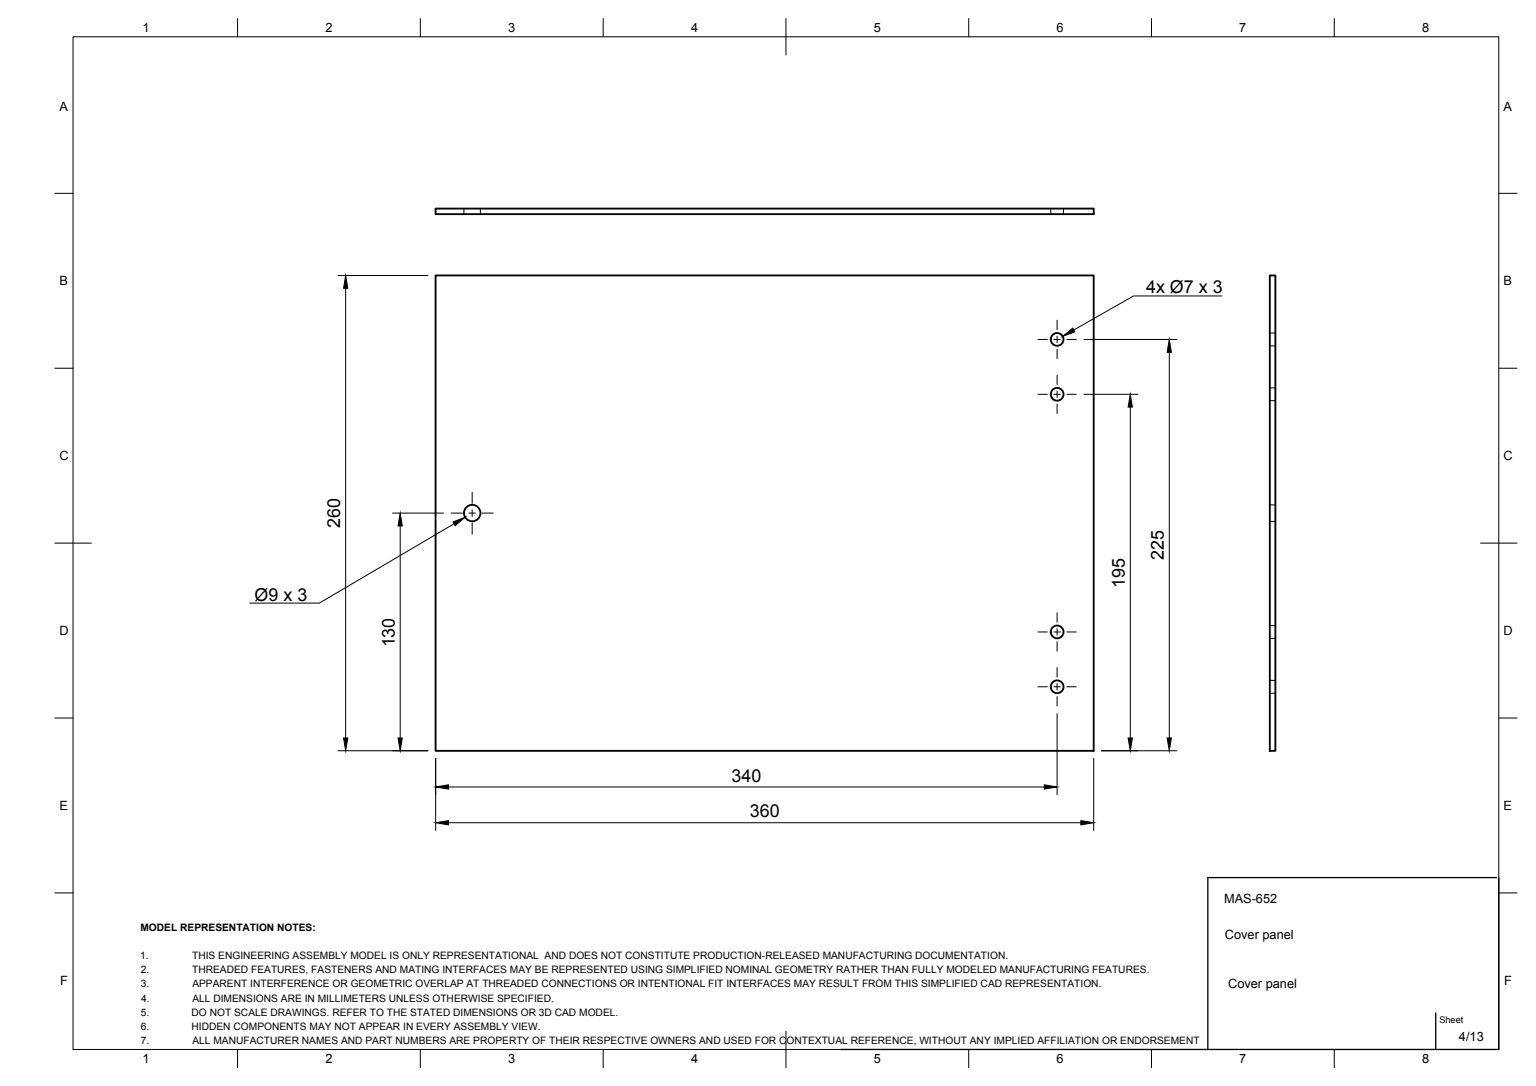
ISO-10303-21;
HEADER;
/* Generated by software containing ST-Developer
 * from STEP Tools, Inc. (www.steptools.com) 
 */

FILE_DESCRIPTION(
/* description */ ('Independent hinged machine back cover with retained hinge pins, perim
eter gasket and quarter-turn cam latch. Nominal cover 360 x 260 x 3 mm
, frame 430 x 300 x 20 mm. No guarding, structural or ingress rating a
ssigned.'),
/* implementation_level */ '2;1');

FILE_NAME(
/* name */ 'Cover panel.step',
/* time_stamp */ '2026-11-09T19:36:59-08:00',
/* author */ (''),
/* organization */ (''),
/* preprocessor_version */ 'ST-DEVELOPER v20.2',
/* originating_system */ 'Autodesk Translation Framework v15.17.0.0',
/* authorisation */ '');

FILE_SCHEMA (('AUTOMOTIVE_DESIGN { 1 0 10303 214 3 1 1 }'));
ENDSEC;

DATA;
#10=MECHANICAL_DESIGN_GEOMETRIC_PRESENTATION_REPRESENTATION('',(#199),#32627);
#163=SHAPE_REPRESENTATION_RELATIONSHIP('SRR','None',#32709,#181);
#181=ADVANCED_BREP_SHAPE_REPRESENTATION('',(#217),#32610);
#199=STYLED_ITEM('',(#32808),#217);
#217=MANIFOLD_SOLID_BREP('Body1',#8676);
#240=FACE_BOUND('',#1113,.T.);
#241=FACE_BOUND('',#1114,.T.);
#242=FACE_BOUND('',#1115,.T.);
#243=FACE_BOUND('',#1116,.T.);
#244=FACE_BOUND('',#1117,.T.);
#245=FACE_BOUND('',#1119,.T.);
#246=FACE_BOUND('',#1120,.T.);
#247=FACE_BOUND('',#1121,.T.);
#248=FACE_BOUND('',#1122,.T.);
#249=FACE_BOUND('',#1123,.T.);
#329=PLANE('',#9096);
#330=PLANE('',#9097);
#331=PLANE('',#9098);
#332=PLANE('',#9099);
#333=PLANE('',#9100);
#334=PLANE('',#9101);
#622=FACE_OUTER_BOUND('',#1103,.T.);
#623=FACE_OUTER_BOUND('',#1104,.T.);
#624=FACE_OUTER_BOUND('',#1105,.T.);
#625=FACE_OUTER_BOUND('',#1106,.T.);
#626=FACE_OUTER_BOUND('',#1107,.T.);
#627=FACE_OUTER_BOUND('',#1108,.T.);
#628=FACE_OUTER_BOUND('',#1109,.T.);
#629=FACE_OUTER_BOUND('',#1110,.T.);
#630=FACE_OUTER_BOUND('',#1111,.T.);
#631=FACE_OUTER_BOUND('',#1112,.T.);
#632=FACE_OUTER_BOUND('',#1118,.T.);
#1103=EDGE_LOOP('',(#6351,#6352,#6353,#6354));
#1104=EDGE_LOOP('',(#6355,#6356,#6357,#6358));
#1105=EDGE_LOOP('',(#6359,#6360,#6361,#6362));
#1106=EDGE_LOOP('',(#6363,#6364,#6365,#6366));
#1107=EDGE_LOOP('',(#6367,#6368,#6369,#6370));
#1108=EDGE_LOOP('',(#6371,#6372,#6373,#6374));
#1109=EDGE_LOOP('',(#6375,#6376,#6377,#6378));
#1110=EDGE_LOOP('',(#6379,#6380,#6381,#6382));
#1111=EDGE_LOOP('',(#6383,#6384,#6385,#6386));
#1112=EDGE_LOOP('',(#6387,#6388,#6389,#6390));
#1113=EDGE_LOOP('',(#6391));
#1114=EDGE_LOOP('',(#6392));
#1115=EDGE_LOOP('',(#6393));
#1116=EDGE_LOOP('',(#6394));
#1117=EDGE_LOOP('',(#6395));
#1118=EDGE_LOOP('',(#6396,#6397,#6398,#6399));
#1119=EDGE_LOOP('',(#6400));
#1120=EDGE_LOOP('',(#6401));
#1121=EDGE_LOOP('',(#6402));
#1122=EDGE_LOOP('',(#6403));
#1123=EDGE_LOOP('',(#6404));
#1485=CIRCLE('',#9082,4.5);
#1486=CIRCLE('',#9083,4.5);
#1487=CIRCLE('',#9085,3.5);
#1488=CIRCLE('',#9086,3.5);
#1489=CIRCLE('',#9088,3.5);
#1490=CIRCLE('',#9089,3.5);
#1491=CIRCLE('',#9091,3.5);
#1492=CIRCLE('',#9092,3.5);
#1493=CIRCLE('',#9094,3.5);
#1494=CIRCLE('',#9095,3.5);
#2339=LINE('',#21642,#2885);
#2340=LINE('',#21648,#2886);
#2341=LINE('',#21654,#2887);
#2342=LINE('',#21660,#2888);
#2343=LINE('',#21666,#2889);
#2344=LINE('',#21671,#2890);
#2345=LINE('',#21673,#2891);
#2346=LINE('',#21675,#2892);
#2347=LINE('',#21676,#2893);
#2348=LINE('',#21679,#2894);
#2349=LINE('',#21681,#2895);
#2350=LINE('',#21682,#2896);
#2351=LINE('',#21685,#2897);
#2352=LINE('',#21687,#2898);
#2353=LINE('',#21688,#2899);
#2354=LINE('',#21690,#2900);
#2355=LINE('',#21691,#2901);
#2885=VECTOR('',#10075,4.5);
#2886=VECTOR('',#10082,3.5);
#2887=VECTOR('',#10089,3.5);
#2888=VECTOR('',#10096,3.5);
#2889=VECTOR('',#10103,3.5);
#2890=VECTOR('',#10108,10.);
#2891=VECTOR('',#10109,10.);
#2892=VECTOR('',#10110,10.);
#2893=VECTOR('',#10111,10.);
#2894=VECTOR('',#10114,10.);
#2895=VECTOR('',#10115,10.);
#2896=VECTOR('',#10116,10.);
#2897=VECTOR('',#10119,10.);
#2898=VECTOR('',#10120,10.);
#2899=VECTOR('',#10121,10.);
#2900=VECTOR('',#10124,10.);
#2901=VECTOR('',#10125,10.);
#3595=VERTEX_POINT('',#21639);
#3596=VERTEX_POINT('',#21641);
#3597=VERTEX_POINT('',#21645);
#3598=VERTEX_POINT('',#21647);
#3599=VERTEX_POINT('',#21651);
#3600=VERTEX_POINT('',#21653);
#3601=VERTEX_POINT('',#21657);
#3602=VERTEX_POINT('',#21659);
#3603=VERTEX_POINT('',#21663);
#3604=VERTEX_POINT('',#21665);
#3605=VERTEX_POINT('',#21669);
#3606=VERTEX_POINT('',#21670);
#3607=VERTEX_POINT('',#21672);
#3608=VERTEX_POINT('',#21674);
#3609=VERTEX_POINT('',#21678);
#3610=VERTEX_POINT('',#21680);
#3611=VERTEX_POINT('',#21684);
#3612=VERTEX_POINT('',#21686);
#4599=EDGE_CURVE('',#3595,#3595,#1485,.T.);
#4600=EDGE_CURVE('',#3595,#3596,#2339,.T.);
#4601=EDGE_CURVE('',#3596,#3596,#1486,.T.);
#4602=EDGE_CURVE('',#3597,#3597,#1487,.T.);
#4603=EDGE_CURVE('',#3597,#3598,#2340,.T.);
#4604=EDGE_CURVE('',#3598,#3598,#1488,.T.);
#4605=EDGE_CURVE('',#3599,#3599,#1489,.T.);
#4606=EDGE_CURVE('',#3599,#3600,#2341,.T.);
#4607=EDGE_CURVE('',#3600,#3600,#1490,.T.);
#4608=EDGE_CURVE('',#3601,#3601,#1491,.T.);
#4609=EDGE_CURVE('',#3601,#3602,#2342,.T.);
#4610=EDGE_CURVE('',#3602,#3602,#1492,.T.);
#4611=EDGE_CURVE('',#3603,#3603,#1493,.T.);
#4612=EDGE_CURVE('',#3603,#3604,#2343,.T.);
#4613=EDGE_CURVE('',#3604,#3604,#1494,.T.);
#4614=EDGE_CURVE('',#3605,#3606,#2344,.T.);
#4615=EDGE_CURVE('',#3606,#3607,#2345,.T.);
#4616=EDGE_CURVE('',#3608,#3607,#2346,.T.);
#4617=EDGE_CURVE('',#3605,#3608,#2347,.T.);
#4618=EDGE_CURVE('',#3609,#3605,#2348,.T.);
#4619=EDGE_CURVE('',#3610,#3608,#2349,.T.);
#4620=EDGE_CURVE('',#3609,#3610,#2350,.T.);
#4621=EDGE_CURVE('',#3611,#3609,#2351,.T.);
#4622=EDGE_CURVE('',#3612,#3610,#2352,.T.);
#4623=EDGE_CURVE('',#3611,#3612,#2353,.T.);
#4624=EDGE_CURVE('',#3606,#3611,#2354,.T.);
#4625=EDGE_CURVE('',#3607,#3612,#2355,.T.);
#6351=ORIENTED_EDGE('',*,*,#4599,.F.);
#6352=ORIENTED_EDGE('',*,*,#4600,.T.);
#6353=ORIENTED_EDGE('',*,*,#4601,.F.);
#6354=ORIENTED_EDGE('',*,*,#4600,.F.);
#6355=ORIENTED_EDGE('',*,*,#4602,.F.);
#6356=ORIENTED_EDGE('',*,*,#4603,.T.);
#6357=ORIENTED_EDGE('',*,*,#4604,.F.);
#6358=ORIENTED_EDGE('',*,*,#4603,.F.);
#6359=ORIENTED_EDGE('',*,*,#4605,.F.);
#6360=ORIENTED_EDGE('',*,*,#4606,.T.);
#6361=ORIENTED_EDGE('',*,*,#4607,.F.);
#6362=ORIENTED_EDGE('',*,*,#4606,.F.);
#6363=ORIENTED_EDGE('',*,*,#4608,.F.);
#6364=ORIENTED_EDGE('',*,*,#4609,.T.);
#6365=ORIENTED_EDGE('',*,*,#4610,.F.);
#6366=ORIENTED_EDGE('',*,*,#4609,.F.);
#6367=ORIENTED_EDGE('',*,*,#4611,.F.);
#6368=ORIENTED_EDGE('',*,*,#4612,.T.);
#6369=ORIENTED_EDGE('',*,*,#4613,.F.);
#6370=ORIENTED_EDGE('',*,*,#4612,.F.);
#6371=ORIENTED_EDGE('',*,*,#4614,.T.);
#6372=ORIENTED_EDGE('',*,*,#4615,.T.);
#6373=ORIENTED_EDGE('',*,*,#4616,.F.);
#6374=ORIENTED_EDGE('',*,*,#4617,.F.);
#6375=ORIENTED_EDGE('',*,*,#4618,.T.);
#6376=ORIENTED_EDGE('',*,*,#4617,.T.);
#6377=ORIENTED_EDGE('',*,*,#4619,.F.);
#6378=ORIENTED_EDGE('',*,*,#4620,.F.);
#6379=ORIENTED_EDGE('',*,*,#4621,.T.);
#6380=ORIENTED_EDGE('',*,*,#4620,.T.);
#6381=ORIENTED_EDGE('',*,*,#4622,.F.);
#6382=ORIENTED_EDGE('',*,*,#4623,.F.);
#6383=ORIENTED_EDGE('',*,*,#4624,.T.);
#6384=ORIENTED_EDGE('',*,*,#4623,.T.);
#6385=ORIENTED_EDGE('',*,*,#4625,.F.);
#6386=ORIENTED_EDGE('',*,*,#4615,.F.);
#6387=ORIENTED_EDGE('',*,*,#4625,.T.);
#6388=ORIENTED_EDGE('',*,*,#4622,.T.);
#6389=ORIENTED_EDGE('',*,*,#4619,.T.);
#6390=ORIENTED_EDGE('',*,*,#4616,.T.);
#6391=ORIENTED_EDGE('',*,*,#4599,.T.);
#6392=ORIENTED_EDGE('',*,*,#4602,.T.);
#6393=ORIENTED_EDGE('',*,*,#4605,.T.);
#6394=ORIENTED_EDGE('',*,*,#4608,.T.);
#6395=ORIENTED_EDGE('',*,*,#4611,.T.);
#6396=ORIENTED_EDGE('',*,*,#4624,.F.);
#6397=ORIENTED_EDGE('',*,*,#4614,.F.);
#6398=ORIENTED_EDGE('',*,*,#4618,.F.);
#6399=ORIENTED_EDGE('',*,*,#4621,.F.);
#6400=ORIENTED_EDGE('',*,*,#4601,.T.);
#6401=ORIENTED_EDGE('',*,*,#4604,.T.);
#6402=ORIENTED_EDGE('',*,*,#4607,.T.);
#6403=ORIENTED_EDGE('',*,*,#4610,.T.);
#6404=ORIENTED_EDGE('',*,*,#4613,.T.);
#8031=CYLINDRICAL_SURFACE('',#9081,4.5);
#8032=CYLINDRICAL_SURFACE('',#9084,3.5);
#8033=CYLINDRICAL_SURFACE('',#9087,3.5);
#8034=CYLINDRICAL_SURFACE('',#9090,3.5);
#8035=CYLINDRICAL_SURFACE('',#9093,3.5);
#8370=ADVANCED_FACE('',(#622),#8031,.F.);
#8371=ADVANCED_FACE('',(#623),#8032,.F.);
#8372=ADVANCED_FACE('',(#624),#8033,.F.);
#8373=ADVANCED_FACE('',(#625),#8034,.F.);
#8374=ADVANCED_FACE('',(#626),#8035,.F.);
#8375=ADVANCED_FACE('',(#627),#329,.T.);
#8376=ADVANCED_FACE('',(#628),#330,.T.);
#8377=ADVANCED_FACE('',(#629),#331,.T.);
#8378=ADVANCED_FACE('',(#630),#332,.T.);
#8379=ADVANCED_FACE('',(#631,#240,#241,#242,#243,#244),#333,.T.);
#8380=ADVANCED_FACE('',(#632,#245,#246,#247,#248,#249),#334,.F.);
#8676=CLOSED_SHELL('',(#8370,#8371,#8372,#8373,#8374,#8375,#8376,#8377,
#8378,#8379,#8380));
#9080=AXIS2_PLACEMENT_3D('',#21637,#10069,#10070);
#9081=AXIS2_PLACEMENT_3D('',#21638,#10071,#10072);
#9082=AXIS2_PLACEMENT_3D('',#21640,#10073,#10074);
#9083=AXIS2_PLACEMENT_3D('',#21643,#10076,#10077);
#9084=AXIS2_PLACEMENT_3D('',#21644,#10078,#10079);
#9085=AXIS2_PLACEMENT_3D('',#21646,#10080,#10081);
#9086=AXIS2_PLACEMENT_3D('',#21649,#10083,#10084);
#9087=AXIS2_PLACEMENT_3D('',#21650,#10085,#10086);
#9088=AXIS2_PLACEMENT_3D('',#21652,#10087,#10088);
#9089=AXIS2_PLACEMENT_3D('',#21655,#10090,#10091);
#9090=AXIS2_PLACEMENT_3D('',#21656,#10092,#10093);
#9091=AXIS2_PLACEMENT_3D('',#21658,#10094,#10095);
#9092=AXIS2_PLACEMENT_3D('',#21661,#10097,#10098);
#9093=AXIS2_PLACEMENT_3D('',#21662,#10099,#10100);
#9094=AXIS2_PLACEMENT_3D('',#21664,#10101,#10102);
#9095=AXIS2_PLACEMENT_3D('',#21667,#10104,#10105);
#9096=AXIS2_PLACEMENT_3D('',#21668,#10106,#10107);
#9097=AXIS2_PLACEMENT_3D('',#21677,#10112,#10113);
#9098=AXIS2_PLACEMENT_3D('',#21683,#10117,#10118);
#9099=AXIS2_PLACEMENT_3D('',#21689,#10122,#10123);
#9100=AXIS2_PLACEMENT_3D('',#21692,#10126,#10127);
#9101=AXIS2_PLACEMENT_3D('',#21693,#10128,#10129);
#10069=DIRECTION('axis',(0.,0.,1.));
#10070=DIRECTION('refdir',(1.,0.,0.));
#10071=DIRECTION('center_axis',(0.,0.,-1.));
#10072=DIRECTION('ref_axis',(1.,0.,0.));
#10073=DIRECTION('center_axis',(0.,0.,-1.));
#10074=DIRECTION('ref_axis',(1.,0.,0.));
#10075=DIRECTION('',(0.,0.,-1.));
#10076=DIRECTION('center_axis',(0.,0.,1.));
#10077=DIRECTION('ref_axis',(1.,0.,0.));
#10078=DIRECTION('center_axis',(0.,0.,-1.));
#10079=DIRECTION('ref_axis',(1.,0.,0.));
#10080=DIRECTION('center_axis',(0.,0.,-1.));
#10081=DIRECTION('ref_axis',(1.,0.,0.));
#10082=DIRECTION('',(0.,0.,-1.));
#10083=DIRECTION('center_axis',(0.,0.,1.));
#10084=DIRECTION('ref_axis',(1.,0.,0.));
#10085=DIRECTION('center_axis',(0.,0.,-1.));
#10086=DIRECTION('ref_axis',(1.,0.,0.));
#10087=DIRECTION('center_axis',(0.,0.,-1.));
#10088=DIRECTION('ref_axis',(1.,0.,0.));
#10089=DIRECTION('',(0.,0.,-1.));
#10090=DIRECTION('center_axis',(0.,0.,1.));
#10091=DIRECTION('ref_axis',(1.,0.,0.));
#10092=DIRECTION('center_axis',(0.,0.,-1.));
#10093=DIRECTION('ref_axis',(1.,0.,0.));
#10094=DIRECTION('center_axis',(0.,0.,-1.));
#10095=DIRECTION('ref_axis',(1.,0.,0.));
#10096=DIRECTION('',(0.,0.,-1.));
#10097=DIRECTION('center_axis',(0.,0.,1.));
#10098=DIRECTION('ref_axis',(1.,0.,0.));
#10099=DIRECTION('center_axis',(0.,0.,-1.));
#10100=DIRECTION('ref_axis',(1.,0.,0.));
#10101=DIRECTION('center_axis',(0.,0.,-1.));
#10102=DIRECTION('ref_axis',(1.,0.,0.));
#10103=DIRECTION('',(0.,0.,-1.));
#10104=DIRECTION('center_axis',(0.,0.,1.));
#10105=DIRECTION('ref_axis',(1.,0.,0.));
#10106=DIRECTION('center_axis',(0.,1.,0.));
#10107=DIRECTION('ref_axis',(-1.,0.,0.));
#10108=DIRECTION('',(-1.,0.,0.));
#10109=DIRECTION('',(0.,0.,1.));
#10110=DIRECTION('',(-1.,0.,0.));
#10111=DIRECTION('',(0.,0.,1.));
#10112=DIRECTION('center_axis',(1.,0.,0.));
#10113=DIRECTION('ref_axis',(0.,1.,0.));
#10114=DIRECTION('',(0.,1.,0.));
#10115=DIRECTION('',(0.,1.,0.));
#10116=DIRECTION('',(0.,0.,1.));
#10117=DIRECTION('center_axis',(0.,-1.,0.));
#10118=DIRECTION('ref_axis',(1.,0.,0.));
#10119=DIRECTION('',(1.,0.,0.));
#10120=DIRECTION('',(1.,0.,0.));
#10121=DIRECTION('',(0.,0.,1.));
#10122=DIRECTION('center_axis',(-1.,0.,0.));
#10123=DIRECTION('ref_axis',(0.,-1.,0.));
#10124=DIRECTION('',(0.,-1.,0.));
#10125=DIRECTION('',(0.,-1.,0.));
#10126=DIRECTION('center_axis',(0.,0.,1.));
#10127=DIRECTION('ref_axis',(1.,0.,0.));
#10128=DIRECTION('center_axis',(0.,0.,1.));
#10129=DIRECTION('ref_axis',(1.,0.,0.));
#21637=CARTESIAN_POINT('',(0.,0.,0.));
#21638=CARTESIAN_POINT('Origin',(160.,0.,1.5));
#21639=CARTESIAN_POINT('',(155.5,5.51091059616309E-16,3.));
#21640=CARTESIAN_POINT('Origin',(160.,0.,3.));
#21641=CARTESIAN_POINT('',(155.5,5.51091059616309E-16,0.));
#21642=CARTESIAN_POINT('',(155.5,5.51091059616309E-16,1.5));
#21643=CARTESIAN_POINT('Origin',(160.,0.,0.));
#21644=CARTESIAN_POINT('Origin',(-160.,65.,1.5));
#21645=CARTESIAN_POINT('',(-163.5,65.,3.));
#21646=CARTESIAN_POINT('Origin',(-160.,65.,3.));
#21647=CARTESIAN_POINT('',(-163.5,65.,0.));
#21648=CARTESIAN_POINT('',(-163.5,65.,1.5));
#21649=CARTESIAN_POINT('Origin',(-160.,65.,0.));
#21650=CARTESIAN_POINT('Origin',(-160.,-95.,1.5));
#21651=CARTESIAN_POINT('',(-163.5,-95.,3.));
#21652=CARTESIAN_POINT('Origin',(-160.,-95.,3.));
#21653=CARTESIAN_POINT('',(-163.5,-95.,0.));
#21654=CARTESIAN_POINT('',(-163.5,-95.,1.5));
#21655=CARTESIAN_POINT('Origin',(-160.,-95.,0.));
#21656=CARTESIAN_POINT('Origin',(-160.,-65.,1.5));
#21657=CARTESIAN_POINT('',(-163.5,-65.,3.));
#21658=CARTESIAN_POINT('Origin',(-160.,-65.,3.));
#21659=CARTESIAN_POINT('',(-163.5,-65.,0.));
#21660=CARTESIAN_POINT('',(-163.5,-65.,1.5));
#21661=CARTESIAN_POINT('Origin',(-160.,-65.,0.));
#21662=CARTESIAN_POINT('Origin',(-160.,95.,1.5));
#21663=CARTESIAN_POINT('',(-163.5,95.,3.));
#21664=CARTESIAN_POINT('Origin',(-160.,95.,3.));
#21665=CARTESIAN_POINT('',(-163.5,95.,0.));
#21666=CARTESIAN_POINT('',(-163.5,95.,1.5));
#21667=CARTESIAN_POINT('Origin',(-160.,95.,0.));
#21668=CARTESIAN_POINT('Origin',(180.,130.,0.));
#21669=CARTESIAN_POINT('',(180.,130.,0.));
#21670=CARTESIAN_POINT('',(-180.,130.,0.));
#21671=CARTESIAN_POINT('',(180.,130.,0.));
#21672=CARTESIAN_POINT('',(-180.,130.,3.));
#21673=CARTESIAN_POINT('',(-180.,130.,0.));
#21674=CARTESIAN_POINT('',(180.,130.,3.));
#21675=CARTESIAN_POINT('',(180.,130.,3.));
#21676=CARTESIAN_POINT('',(180.,130.,0.));
#21677=CARTESIAN_POINT('Origin',(180.,-130.,0.));
#21678=CARTESIAN_POINT('',(180.,-130.,0.));
#21679=CARTESIAN_POINT('',(180.,-130.,0.));
#21680=CARTESIAN_POINT('',(180.,-130.,3.));
#21681=CARTESIAN_POINT('',(180.,-130.,3.));
#21682=CARTESIAN_POINT('',(180.,-130.,0.));
#21683=CARTESIAN_POINT('Origin',(-180.,-130.,0.));
#21684=CARTESIAN_POINT('',(-180.,-130.,0.));
#21685=CARTESIAN_POINT('',(-180.,-130.,0.));
#21686=CARTESIAN_POINT('',(-180.,-130.,3.));
#21687=CARTESIAN_POINT('',(-180.,-130.,3.));
#21688=CARTESIAN_POINT('',(-180.,-130.,0.));
#21689=CARTESIAN_POINT('Origin',(-180.,130.,0.));
#21690=CARTESIAN_POINT('',(-180.,130.,0.));
#21691=CARTESIAN_POINT('',(-180.,130.,3.));
#21692=CARTESIAN_POINT('Origin',(0.,0.,3.));
#21693=CARTESIAN_POINT('Origin',(0.,0.,0.));
#32590=UNCERTAINTY_MEASURE_WITH_UNIT(LENGTH_MEASURE(0.01),#32628,
'DISTANCE_ACCURACY_VALUE',
'Maximum model space distance between geometric entities at asserted c
onnectivities');
#32607=UNCERTAINTY_MEASURE_WITH_UNIT(LENGTH_MEASURE(0.01),#32628,
'DISTANCE_ACCURACY_VALUE',
'Maximum model space distance between geometric entities at asserted c
onnectivities');
#32610=(
GEOMETRIC_REPRESENTATION_CONTEXT(3)
GLOBAL_UNCERTAINTY_ASSIGNED_CONTEXT((#32590))
GLOBAL_UNIT_ASSIGNED_CONTEXT((#32628,#32630,#32631))
REPRESENTATION_CONTEXT('','3D')
);
#32627=(
GEOMETRIC_REPRESENTATION_CONTEXT(3)
GLOBAL_UNCERTAINTY_ASSIGNED_CONTEXT((#32607))
GLOBAL_UNIT_ASSIGNED_CONTEXT((#32628,#32630,#32631))
REPRESENTATION_CONTEXT('','3D')
);
#32628=(
LENGTH_UNIT()
NAMED_UNIT(*)
SI_UNIT(.MILLI.,.METRE.)
);
#32630=(
NAMED_UNIT(*)
PLANE_ANGLE_UNIT()
SI_UNIT($,.RADIAN.)
);
#32631=(
NAMED_UNIT(*)
SI_UNIT($,.STERADIAN.)
SOLID_ANGLE_UNIT()
);
#32634=SHAPE_DEFINITION_REPRESENTATION(#32653,#32709);
#32653=PRODUCT_DEFINITION_SHAPE('',$,#32729);
#32709=SHAPE_REPRESENTATION('',(#9080),#32610);
#32726=PRODUCT_DEFINITION_CONTEXT('part definition',#32785,'design');
#32729=PRODUCT_DEFINITION('Cover panel','Cover panel',#32748,#32726);
#32748=PRODUCT_DEFINITION_FORMATION('',$,#32789);
#32785=APPLICATION_CONTEXT(
'Core Data for Automotive Mechanical Design Process');
#32786=PRODUCT_CONTEXT('part definition',#32785,'mechanical');
#32789=PRODUCT('Cover panel','Cover panel',$,(#32786));
#32808=PRESENTATION_STYLE_ASSIGNMENT((#32815));
#32815=SURFACE_STYLE_USAGE(.BOTH.,#32822);
#32822=SURFACE_SIDE_STYLE('',(#32829));
#32829=SURFACE_STYLE_FILL_AREA(#32836);
#32836=FILL_AREA_STYLE('Light blue',(#32843));
#32843=FILL_AREA_STYLE_COLOUR('Light blue',#32850);
#32850=COLOUR_RGB('Light blue',0.662745098039216,0.831372549019608,0.949019607843137);
ENDSEC;
END-ISO-10303-21;
